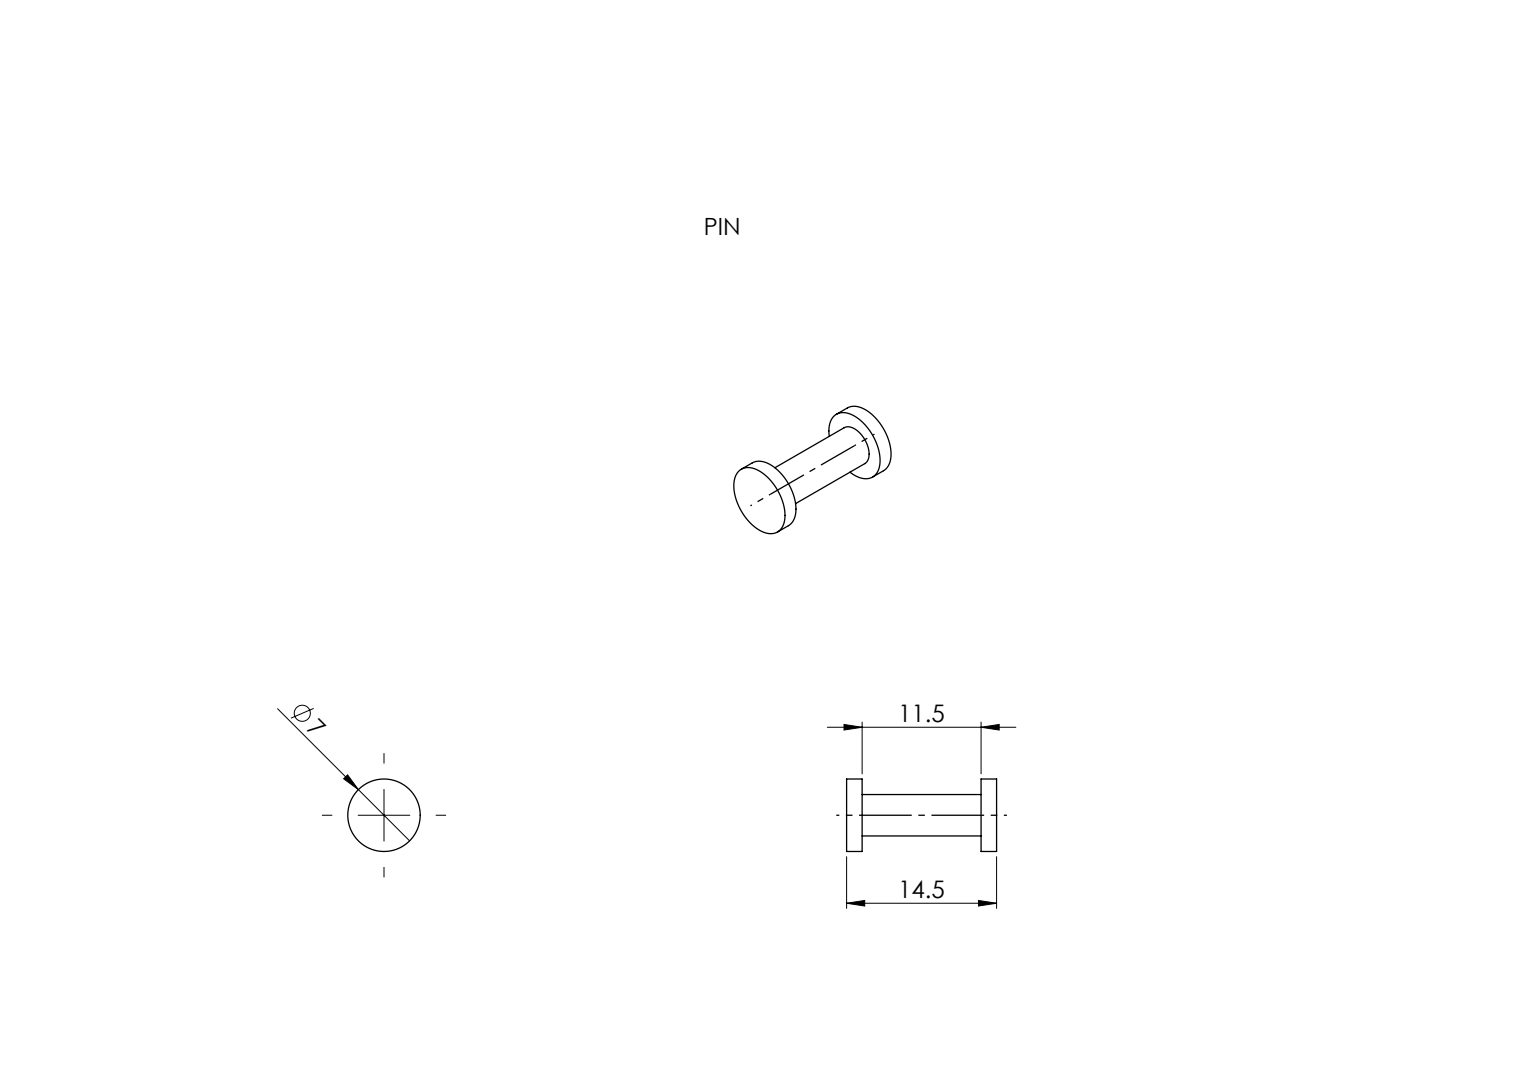
ISO-10303-21;
HEADER;
FILE_DESCRIPTION (('STEP AP214'),
    '1' );
FILE_NAME ('pin.step',
    '2026-10-08T13:56:24',
    ( '' ),
    ( '' ),
    'SwSTEP 2.0',
    'SolidWorks 2026',
    '' );
FILE_SCHEMA (( 'AUTOMOTIVE_DESIGN' ));
ENDSEC;

DATA;
#12=DIRECTION ( 'NONE',  ( 0.000000000000000000, 0.000000000000000000, 1.000000000000000000 ) ) ;
#38=ORIENTED_EDGE ( 'NONE', *, *, #402, .T. ) ;
#114=STYLED_ITEM ( 'NONE', ( #1544 ), #1156 ) ;
#128=FACE_OUTER_BOUND ( 'NONE', #6380, .T. ) ;
#244=CIRCLE ( 'NONE', #13904, 3.499999999999999556 ) ;
#268=ORIENTED_EDGE ( 'NONE', *, *, #2450, .T. ) ;
#279=SHAPE_REPRESENTATION ( 'pin', ( #3223 ), #1392 ) ;
#300=DIRECTION ( 'NONE',  ( 1.000000000000000000, 0.000000000000000000, 0.000000000000000000 ) ) ;
#402=EDGE_CURVE ( 'NONE', #3787, #10893, #14404, .T. ) ;
#420=ORIENTED_EDGE ( 'NONE', *, *, #9806, .F. ) ;
#470=AXIS2_PLACEMENT_3D ( 'NONE', #10148, #3841, #13765 ) ;
#493=AXIS2_PLACEMENT_3D ( 'NONE', #9026, #13762, #300 ) ;
#510=CYLINDRICAL_SURFACE ( 'NONE', #2443, 3.499999999999999556 ) ;
#545=ORIENTED_EDGE ( 'NONE', *, *, #14696, .T. ) ;
#561=ORIENTED_EDGE ( 'NONE', *, *, #4255, .T. ) ;
#598=ORIENTED_EDGE ( 'NONE', *, *, #1280, .F. ) ;
#604=CIRCLE ( 'NONE', #12193, 3.499999999999999556 ) ;
#652=DIRECTION ( 'NONE',  ( 0.000000000000000000, 0.000000000000000000, -1.000000000000000000 ) ) ;
#744=AXIS2_PLACEMENT_3D ( 'NONE', #6292, #7508, #3860 ) ;
#761=DIRECTION ( 'NONE',  ( 1.000000000000000000, 0.000000000000000000, 0.000000000000000000 ) ) ;
#824=PRESENTATION_STYLE_ASSIGNMENT (( #8512 ) ) ;
#867=EDGE_CURVE ( 'NONE', #14345, #10556, #6652, .T. ) ;
#971=FACE_OUTER_BOUND ( 'NONE', #5873, .T. ) ;
#1022=CARTESIAN_POINT ( 'NONE',  ( 16.49999999999956657, -8.786575603324269439E-13, 1.500000000000000000 ) ) ;
#1029=FACE_BOUND ( 'NONE', #10956, .T. ) ;
#1124=DIRECTION ( 'NONE',  ( 1.000000000000000000, 0.000000000000000000, -0.000000000000000000 ) ) ;
#1156=ADVANCED_BREP_SHAPE_REPRESENTATION ( '', ( #14368, #3223 ), #1392 ) ;
#1214=VERTEX_POINT ( 'NONE', #3633 ) ;
#1279=DIRECTION ( 'NONE',  ( 1.000000000000000000, 0.000000000000000000, 0.000000000000000000 ) ) ;
#1280=EDGE_CURVE ( 'NONE', #14345, #6321, #604, .T. ) ;
#1287=DIRECTION ( 'NONE',  ( 0.000000000000000000, 0.000000000000000000, 1.000000000000000000 ) ) ;
#1293=ORIENTED_EDGE ( 'NONE', *, *, #14089, .T. ) ;
#1392=( GEOMETRIC_REPRESENTATION_CONTEXT ( 3 ) GLOBAL_UNCERTAINTY_ASSIGNED_CONTEXT ( ( #13859 ) ) GLOBAL_UNIT_ASSIGNED_CONTEXT ( ( #13328, #11002, #7290 ) ) REPRESENTATION_CONTEXT ( 'NONE', 'WORKASPACE' ) );
#1399=EDGE_CURVE ( 'NONE', #3787, #13461, #8894, .T. ) ;
#1418=DIRECTION ( 'NONE',  ( -0.000000000000000000, -0.000000000000000000, 1.000000000000000000 ) ) ;
#1458=FACE_OUTER_BOUND ( 'NONE', #4862, .T. ) ;
#1544=PRESENTATION_STYLE_ASSIGNMENT (( #6858 ) ) ;
#1546=DIRECTION ( 'NONE',  ( -0.000000000000000000, -0.000000000000000000, -1.000000000000000000 ) ) ;
#1885=DIRECTION ( 'NONE',  ( 0.000000000000000000, 0.000000000000000000, 1.000000000000000000 ) ) ;
#1897=ADVANCED_FACE ( 'NONE', ( #3041 ), #4340, .T. ) ;
#1912=SURFACE_SIDE_STYLE ('',( #4264 ) ) ;
#2171=CARTESIAN_POINT ( 'NONE',  ( 19.99999999999956657, -8.786575603324269439E-13, -13.00000000000000000 ) ) ;
#2257=DIRECTION ( 'NONE',  ( -1.000000000000000000, 0.000000000000000000, 0.000000000000000000 ) ) ;
#2264=( NAMED_UNIT ( * ) SI_UNIT ( $, .STERADIAN. ) SOLID_ANGLE_UNIT ( ) );
#2282=PRODUCT ( 'pin', 'pin', '', ( #8596 ) ) ;
#2424=SHAPE_DEFINITION_REPRESENTATION ( #11948, #279 ) ;
#2431=AXIS2_PLACEMENT_3D ( 'NONE', #12948, #1885, #6826 ) ;
#2443=AXIS2_PLACEMENT_3D ( 'NONE', #2666, #1546, #7617 ) ;
#2450=EDGE_CURVE ( 'NONE', #10893, #1214, #15851, .T. ) ;
#2467=ADVANCED_FACE ( 'NONE', ( #14632, #8508 ), #7283, .F. ) ;
#2621=VERTEX_POINT ( 'NONE', #14297 ) ;
#2664=FILL_AREA_STYLE_COLOUR ( '', #3713 ) ;
#2666=CARTESIAN_POINT ( 'NONE',  ( 19.99999999999956657, -8.786575603324269439E-13, 1.500000000000000000 ) ) ;
#2707=COLOUR_RGB ( '', 0.72549020, 0.75294118, 0.79215686) ;
#2730=DIRECTION ( 'NONE',  ( -1.000000000000000000, 0.000000000000000000, 0.000000000000000000 ) ) ;
#2733=DIRECTION ( 'NONE',  ( 0.000000000000000000, 0.000000000000000000, 1.000000000000000000 ) ) ;
#2775=CIRCLE ( 'NONE', #12586, 3.499999999999999556 ) ;
#2780=APPLICATION_CONTEXT ( 'automotive_design' ) ;
#2797=CIRCLE ( 'NONE', #13897, 1.999999999999998224 ) ;
#2804=DIRECTION ( 'NONE',  ( 0.000000000000000000, 0.000000000000000000, 1.000000000000000000 ) ) ;
#2857=ORIENTED_EDGE ( 'NONE', *, *, #14089, .F. ) ;
#2908=DIRECTION ( 'NONE',  ( 0.000000000000000000, 0.000000000000000000, 1.000000000000000000 ) ) ;
#2968=CIRCLE ( 'NONE', #11735, 3.499999999999999556 ) ;
#3041=FACE_OUTER_BOUND ( 'NONE', #8493, .T. ) ;
#3057=( NAMED_UNIT ( * ) PLANE_ANGLE_UNIT ( ) SI_UNIT ( $, .RADIAN. ) );
#3115=EDGE_LOOP ( 'NONE', ( #5621, #10954 ) ) ;
#3133=VERTEX_POINT ( 'NONE', #5634 ) ;
#3171=VERTEX_POINT ( 'NONE', #11913 ) ;
#3223=AXIS2_PLACEMENT_3D ( 'NONE', #11897, #11972, #4638 ) ;
#3330=SURFACE_SIDE_STYLE ('',( #15617 ) ) ;
#3377=DIRECTION ( 'NONE',  ( 1.000000000000000000, 0.000000000000000000, 0.000000000000000000 ) ) ;
#3390=CARTESIAN_POINT ( 'NONE',  ( 19.99999999999956657, -8.786575603324269439E-13, 1.500000000000000000 ) ) ;
#3458=MECHANICAL_DESIGN_GEOMETRIC_PRESENTATION_REPRESENTATION('',(#114),#10179);
#3461=AXIS2_PLACEMENT_3D ( 'NONE', #12185, #1287, #1124 ) ;
#3471=( NAMED_UNIT ( * ) PLANE_ANGLE_UNIT ( ) SI_UNIT ( $, .RADIAN. ) );
#3501=CARTESIAN_POINT ( 'NONE',  ( 19.99999999999956657, -8.786575603324269439E-13, -11.50000000000000000 ) ) ;
#3633=CARTESIAN_POINT ( 'NONE',  ( 17.99999999999957012, -8.784126309725975241E-13, 0.000000000000000000 ) ) ;
#3688=DIRECTION ( 'NONE',  ( 0.000000000000000000, 0.000000000000000000, 1.000000000000000000 ) ) ;
#3702=DIRECTION ( 'NONE',  ( 1.000000000000000000, 0.000000000000000000, -0.000000000000000000 ) ) ;
#3713=COLOUR_RGB ( '', 0.72549020, 0.75294118, 0.79215686) ;
#3724=CARTESIAN_POINT ( 'NONE',  ( 19.99999999999956657, -8.786575603324269439E-13, -13.00000000000000000 ) ) ;
#3734=ORIENTED_EDGE ( 'NONE', *, *, #14085, .T. ) ;
#3787=VERTEX_POINT ( 'NONE', #14980 ) ;
#3835=VECTOR ( 'NONE', #8593, 1000.000000000000000 ) ;
#3841=DIRECTION ( 'NONE',  ( -0.000000000000000000, -0.000000000000000000, -1.000000000000000000 ) ) ;
#3860=DIRECTION ( 'NONE',  ( 1.000000000000000000, 0.000000000000000000, 0.000000000000000000 ) ) ;
#4016=AXIS2_PLACEMENT_3D ( 'NONE', #2171, #8417, #1279 ) ;
#4126=EDGE_LOOP ( 'NONE', ( #598, #10600, #4186, #11155 ) ) ;
#4148=PRODUCT_DEFINITION_CONTEXT ( 'detailed design', #2780, 'design' ) ;
#4186=ORIENTED_EDGE ( 'NONE', *, *, #9806, .T. ) ;
#4255=EDGE_CURVE ( 'NONE', #13119, #10556, #13568, .T. ) ;
#4264=SURFACE_STYLE_FILL_AREA ( #7536 ) ;
#4340=CYLINDRICAL_SURFACE ( 'NONE', #7830, 1.999999999999998224 ) ;
#4360=ADVANCED_FACE ( 'NONE', ( #1029, #12326 ), #5964, .F. ) ;
#4374=ORIENTED_EDGE ( 'NONE', *, *, #7133, .T. ) ;
#4468=CARTESIAN_POINT ( 'NONE',  ( 16.49999999999956657, -8.786575603324269439E-13, 1.500000000000000000 ) ) ;
#4638=DIRECTION ( 'NONE',  ( 1.000000000000000000, 0.000000000000000000, 0.000000000000000000 ) ) ;
#4640=ORIENTED_EDGE ( 'NONE', *, *, #4912, .F. ) ;
#4744=CARTESIAN_POINT ( 'NONE',  ( 19.99999999999956657, -8.786575603324269439E-13, -11.50000000000000000 ) ) ;
#4827=CARTESIAN_POINT ( 'NONE',  ( 19.99999999999956657, -8.786575603324269439E-13, -11.50000000000000000 ) ) ;
#4862=EDGE_LOOP ( 'NONE', ( #9433, #4374, #9993, #8827 ) ) ;
#4902=EDGE_LOOP ( 'NONE', ( #6854, #14386 ) ) ;
#4906=DIRECTION ( 'NONE',  ( 0.000000000000000000, 0.000000000000000000, -1.000000000000000000 ) ) ;
#4912=EDGE_CURVE ( 'NONE', #10893, #3787, #8460, .T. ) ;
#5022=LINE ( 'NONE', #13484, #3835 ) ;
#5101=( NAMED_UNIT ( * ) SI_UNIT ( $, .STERADIAN. ) SOLID_ANGLE_UNIT ( ) );
#5151=DIRECTION ( 'NONE',  ( 0.000000000000000000, 0.000000000000000000, 1.000000000000000000 ) ) ;
#5508=ORIENTED_EDGE ( 'NONE', *, *, #7307, .F. ) ;
#5576=DIRECTION ( 'NONE',  ( -1.000000000000000000, 0.000000000000000000, 0.000000000000000000 ) ) ;
#5621=ORIENTED_EDGE ( 'NONE', *, *, #8865, .F. ) ;
#5634=CARTESIAN_POINT ( 'NONE',  ( 23.49999999999956657, -8.782289339527253835E-13, 1.500000000000000000 ) ) ;
#5873=EDGE_LOOP ( 'NONE', ( #1293, #545 ) ) ;
#5964=PLANE ( 'NONE',  #12294 ) ;
#6005=ADVANCED_FACE ( 'NONE', ( #8859 ), #6589, .T. ) ;
#6166=PLANE ( 'NONE',  #8962 ) ;
#6209=DIRECTION ( 'NONE',  ( -1.000000000000000000, 0.000000000000000000, 0.000000000000000000 ) ) ;
#6225=FACE_OUTER_BOUND ( 'NONE', #4126, .T. ) ;
#6292=CARTESIAN_POINT ( 'NONE',  ( 19.99999999999956657, -8.786575603324269439E-13, 0.000000000000000000 ) ) ;
#6320=CARTESIAN_POINT ( 'NONE',  ( 19.99999999999956657, -8.786575603324269439E-13, 0.000000000000000000 ) ) ;
#6321=VERTEX_POINT ( 'NONE', #14810 ) ;
#6380=EDGE_LOOP ( 'NONE', ( #8663, #11359, #11699, #561 ) ) ;
#6403=ORIENTED_EDGE ( 'NONE', *, *, #8676, .T. ) ;
#6481=( LENGTH_UNIT ( ) NAMED_UNIT ( * ) SI_UNIT ( .MILLI., .METRE. ) );
#6521=CARTESIAN_POINT ( 'NONE',  ( 23.49999999999956657, -8.786575603324269439E-13, -13.00000000000000000 ) ) ;
#6589=CYLINDRICAL_SURFACE ( 'NONE', #470, 3.499999999999999556 ) ;
#6652=LINE ( 'NONE', #8997, #15308 ) ;
#6732=ORIENTED_EDGE ( 'NONE', *, *, #1399, .T. ) ;
#6767=DIRECTION ( 'NONE',  ( 1.000000000000000000, 0.000000000000000000, 0.000000000000000000 ) ) ;
#6821=DIRECTION ( 'NONE',  ( 0.000000000000000000, 0.000000000000000000, 1.000000000000000000 ) ) ;
#6826=DIRECTION ( 'NONE',  ( 1.000000000000000000, 0.000000000000000000, 0.000000000000000000 ) ) ;
#6835=VECTOR ( 'NONE', #12, 1000.000000000000000 ) ;
#6854=ORIENTED_EDGE ( 'NONE', *, *, #7307, .T. ) ;
#6858=SURFACE_STYLE_USAGE ( .BOTH. , #1912 ) ;
#6874=AXIS2_PLACEMENT_3D ( 'NONE', #3390, #15842, #3702 ) ;
#7006=EDGE_CURVE ( 'NONE', #1214, #13461, #2797, .T. ) ;
#7008=DIRECTION ( 'NONE',  ( 0.000000000000000000, 0.000000000000000000, 1.000000000000000000 ) ) ;
#7112=CIRCLE ( 'NONE', #2431, 3.499999999999999556 ) ;
#7120=PLANE ( 'NONE',  #6874 ) ;
#7133=EDGE_CURVE ( 'NONE', #3133, #3171, #5022, .T. ) ;
#7283=PLANE ( 'NONE',  #3461 ) ;
#7290=( NAMED_UNIT ( * ) SI_UNIT ( $, .STERADIAN. ) SOLID_ANGLE_UNIT ( ) );
#7307=EDGE_CURVE ( 'NONE', #13461, #1214, #10305, .T. ) ;
#7442=DIRECTION ( 'NONE',  ( 0.000000000000000000, 0.000000000000000000, -1.000000000000000000 ) ) ;
#7508=DIRECTION ( 'NONE',  ( 0.000000000000000000, 0.000000000000000000, 1.000000000000000000 ) ) ;
#7536=FILL_AREA_STYLE ('',( #2664 ) ) ;
#7617=DIRECTION ( 'NONE',  ( -1.000000000000000000, 0.000000000000000000, 0.000000000000000000 ) ) ;
#7655=ORIENTED_EDGE ( 'NONE', *, *, #1280, .T. ) ;
#7830=AXIS2_PLACEMENT_3D ( 'NONE', #13043, #7008, #6767 ) ;
#7897=CARTESIAN_POINT ( 'NONE',  ( 19.99999999999956657, -8.786575603324269439E-13, -11.50000000000000000 ) ) ;
#7961=LINE ( 'NONE', #4468, #8160 ) ;
#8160=VECTOR ( 'NONE', #10544, 1000.000000000000000 ) ;
#8186=CLOSED_SHELL ( 'NONE', ( #11457, #11195, #1897, #8884, #6005, #11456, #2467, #9196, #12602, #4360 ) ) ;
#8379=DIRECTION ( 'NONE',  ( 1.000000000000000000, 0.000000000000000000, 0.000000000000000000 ) ) ;
#8417=DIRECTION ( 'NONE',  ( -0.000000000000000000, -0.000000000000000000, 1.000000000000000000 ) ) ;
#8460=CIRCLE ( 'NONE', #9479, 1.999999999999998224 ) ;
#8493=EDGE_LOOP ( 'NONE', ( #38, #268, #5508, #11280 ) ) ;
#8508=FACE_OUTER_BOUND ( 'NONE', #3115, .T. ) ;
#8512=SURFACE_STYLE_USAGE ( .BOTH. , #3330 ) ;
#8593=DIRECTION ( 'NONE',  ( -0.000000000000000000, -0.000000000000000000, -1.000000000000000000 ) ) ;
#8596=PRODUCT_CONTEXT ( 'NONE', #14240, 'mechanical' ) ;
#8633=DIRECTION ( 'NONE',  ( 0.000000000000000000, 0.000000000000000000, -1.000000000000000000 ) ) ;
#8663=ORIENTED_EDGE ( 'NONE', *, *, #867, .F. ) ;
#8676=EDGE_CURVE ( 'NONE', #6321, #14345, #2775, .T. ) ;
#8719=FACE_OUTER_BOUND ( 'NONE', #14361, .T. ) ;
#8827=ORIENTED_EDGE ( 'NONE', *, *, #14085, .F. ) ;
#8859=FACE_OUTER_BOUND ( 'NONE', #11536, .T. ) ;
#8865=EDGE_CURVE ( 'NONE', #2621, #3171, #13356, .T. ) ;
#8884=ADVANCED_FACE ( 'NONE', ( #8719 ), #13625, .T. ) ;
#8894=LINE ( 'NONE', #13796, #15576 ) ;
#8962=AXIS2_PLACEMENT_3D ( 'NONE', #3724, #14431, #13192 ) ;
#8997=CARTESIAN_POINT ( 'NONE',  ( 16.49999999999956657, -8.782289339527253835E-13, -13.00000000000000000 ) ) ;
#9026=CARTESIAN_POINT ( 'NONE',  ( 19.99999999999956657, -8.786575603324269439E-13, -13.00000000000000000 ) ) ;
#9092=CARTESIAN_POINT ( 'NONE',  ( 19.99999999999956657, -8.786575603324269439E-13, 1.500000000000000000 ) ) ;
#9126=ORIENTED_EDGE ( 'NONE', *, *, #8865, .T. ) ;
#9173=STYLED_ITEM ( 'NONE', ( #824 ), #14368 ) ;
#9196=ADVANCED_FACE ( 'NONE', ( #128 ), #11112, .T. ) ;
#9220=CARTESIAN_POINT ( 'NONE',  ( 19.99999999999956657, -8.786575603324269439E-13, -13.00000000000000000 ) ) ;
#9304=EDGE_LOOP ( 'NONE', ( #13905, #420 ) ) ;
#9393=FILL_AREA_STYLE_COLOUR ( '', #2707 ) ;
#9433=ORIENTED_EDGE ( 'NONE', *, *, #14696, .F. ) ;
#9468=AXIS2_PLACEMENT_3D ( 'NONE', #4827, #8633, #6209 ) ;
#9479=AXIS2_PLACEMENT_3D ( 'NONE', #3501, #9730, #8379 ) ;
#9690=DIRECTION ( 'NONE',  ( 0.000000000000000000, 0.000000000000000000, -1.000000000000000000 ) ) ;
#9730=DIRECTION ( 'NONE',  ( 0.000000000000000000, 0.000000000000000000, 1.000000000000000000 ) ) ;
#9794=ORIENTED_EDGE ( 'NONE', *, *, #2450, .F. ) ;
#9806=EDGE_CURVE ( 'NONE', #10556, #13119, #244, .T. ) ;
#9989=PRODUCT_DEFINITION_FORMATION_WITH_SPECIFIED_SOURCE ( 'ANY', '', #2282, .NOT_KNOWN. ) ;
#9993=ORIENTED_EDGE ( 'NONE', *, *, #11179, .T. ) ;
#10026=CARTESIAN_POINT ( 'NONE',  ( 17.99999999999957012, -8.784126309725975241E-13, -11.50000000000000000 ) ) ;
#10080=DIRECTION ( 'NONE',  ( 1.000000000000000000, 0.000000000000000000, 0.000000000000000000 ) ) ;
#10119=DIRECTION ( 'NONE',  ( -0.000000000000000000, -0.000000000000000000, 1.000000000000000000 ) ) ;
#10148=CARTESIAN_POINT ( 'NONE',  ( 19.99999999999956657, -8.786575603324269439E-13, 1.500000000000000000 ) ) ;
#10179=( GEOMETRIC_REPRESENTATION_CONTEXT ( 3 ) GLOBAL_UNCERTAINTY_ASSIGNED_CONTEXT ( ( #12702 ) ) GLOBAL_UNIT_ASSIGNED_CONTEXT ( ( #6481, #3057, #5101 ) ) REPRESENTATION_CONTEXT ( 'NONE', 'WORKASPACE' ) );
#10182=CARTESIAN_POINT ( 'NONE',  ( 19.99999999999956657, -8.786575603324269439E-13, -11.50000000000000000 ) ) ;
#10285=DIRECTION ( 'NONE',  ( 1.000000000000000000, 0.000000000000000000, 0.000000000000000000 ) ) ;
#10305=CIRCLE ( 'NONE', #14687, 1.999999999999998224 ) ;
#10410=ORIENTED_EDGE ( 'NONE', *, *, #402, .F. ) ;
#10544=DIRECTION ( 'NONE',  ( -0.000000000000000000, -0.000000000000000000, -1.000000000000000000 ) ) ;
#10556=VERTEX_POINT ( 'NONE', #15643 ) ;
#10600=ORIENTED_EDGE ( 'NONE', *, *, #867, .T. ) ;
#10893=VERTEX_POINT ( 'NONE', #14250 ) ;
#10912=FILL_AREA_STYLE ('',( #9393 ) ) ;
#10954=ORIENTED_EDGE ( 'NONE', *, *, #11179, .F. ) ;
#10956=EDGE_LOOP ( 'NONE', ( #10410, #4640 ) ) ;
#10967=CARTESIAN_POINT ( 'NONE',  ( 19.99999999999956657, -8.786575603324269439E-13, 0.000000000000000000 ) ) ;
#10976=MECHANICAL_DESIGN_GEOMETRIC_PRESENTATION_REPRESENTATION('',(#9173),#11981);
#11002=( NAMED_UNIT ( * ) PLANE_ANGLE_UNIT ( ) SI_UNIT ( $, .RADIAN. ) );
#11112=CYLINDRICAL_SURFACE ( 'NONE', #493, 3.499999999999999556 ) ;
#11155=ORIENTED_EDGE ( 'NONE', *, *, #13618, .F. ) ;
#11179=EDGE_CURVE ( 'NONE', #3171, #2621, #12772, .T. ) ;
#11195=ADVANCED_FACE ( 'NONE', ( #1458 ), #510, .T. ) ;
#11280=ORIENTED_EDGE ( 'NONE', *, *, #1399, .F. ) ;
#11359=ORIENTED_EDGE ( 'NONE', *, *, #8676, .F. ) ;
#11456=ADVANCED_FACE ( 'NONE', ( #971 ), #7120, .T. ) ;
#11457=ADVANCED_FACE ( 'NONE', ( #6225 ), #13231, .T. ) ;
#11536=EDGE_LOOP ( 'NONE', ( #13078, #2857, #3734, #9126 ) ) ;
#11628=EDGE_LOOP ( 'NONE', ( #6403, #7655 ) ) ;
#11699=ORIENTED_EDGE ( 'NONE', *, *, #13618, .T. ) ;
#11726=VECTOR ( 'NONE', #1418, 1000.000000000000000 ) ;
#11735=AXIS2_PLACEMENT_3D ( 'NONE', #9092, #13018, #761 ) ;
#11897=CARTESIAN_POINT ( 'NONE',  ( 0.000000000000000000, 0.000000000000000000, 0.000000000000000000 ) ) ;
#11913=CARTESIAN_POINT ( 'NONE',  ( 23.49999999999956657, -8.782289339527253835E-13, 0.000000000000000000 ) ) ;
#11948=PRODUCT_DEFINITION_SHAPE ( 'NONE', 'NONE',  #13413 ) ;
#11972=DIRECTION ( 'NONE',  ( 0.000000000000000000, 0.000000000000000000, 1.000000000000000000 ) ) ;
#11981=( GEOMETRIC_REPRESENTATION_CONTEXT ( 3 ) GLOBAL_UNCERTAINTY_ASSIGNED_CONTEXT ( ( #15507 ) ) GLOBAL_UNIT_ASSIGNED_CONTEXT ( ( #15700, #3471, #2264 ) ) REPRESENTATION_CONTEXT ( 'NONE', 'WORKASPACE' ) );
#12004=CARTESIAN_POINT ( 'NONE',  ( 21.99999999999956657, -8.786575603324269439E-13, 0.000000000000000000 ) ) ;
#12185=CARTESIAN_POINT ( 'NONE',  ( 19.99999999999956657, -8.786575603324269439E-13, 0.000000000000000000 ) ) ;
#12193=AXIS2_PLACEMENT_3D ( 'NONE', #13315, #9690, #2257 ) ;
#12294=AXIS2_PLACEMENT_3D ( 'NONE', #4744, #4906, #13378 ) ;
#12326=FACE_OUTER_BOUND ( 'NONE', #9304, .T. ) ;
#12439=ORIENTED_EDGE ( 'NONE', *, *, #4912, .T. ) ;
#12586=AXIS2_PLACEMENT_3D ( 'NONE', #9220, #652, #5576 ) ;
#12602=ADVANCED_FACE ( 'NONE', ( #15647 ), #6166, .T. ) ;
#12645=LINE ( 'NONE', #6521, #11726 ) ;
#12702=UNCERTAINTY_MEASURE_WITH_UNIT (LENGTH_MEASURE( 1.000000000000000082E-05 ), #6481, 'distance_accuracy_value', 'NONE');
#12772=CIRCLE ( 'NONE', #13540, 3.499999999999999556 ) ;
#12948=CARTESIAN_POINT ( 'NONE',  ( 19.99999999999956657, -8.786575603324269439E-13, 1.500000000000000000 ) ) ;
#13018=DIRECTION ( 'NONE',  ( 0.000000000000000000, 0.000000000000000000, 1.000000000000000000 ) ) ;
#13043=CARTESIAN_POINT ( 'NONE',  ( 19.99999999999956657, -8.786575603324269439E-13, -11.50000000000000000 ) ) ;
#13078=ORIENTED_EDGE ( 'NONE', *, *, #7133, .F. ) ;
#13103=DIRECTION ( 'NONE',  ( 1.000000000000000000, 0.000000000000000000, 0.000000000000000000 ) ) ;
#13119=VERTEX_POINT ( 'NONE', #13638 ) ;
#13192=DIRECTION ( 'NONE',  ( -1.000000000000000000, 0.000000000000000000, -0.000000000000000000 ) ) ;
#13231=CYLINDRICAL_SURFACE ( 'NONE', #4016, 3.499999999999999556 ) ;
#13315=CARTESIAN_POINT ( 'NONE',  ( 19.99999999999956657, -8.786575603324269439E-13, -13.00000000000000000 ) ) ;
#13328=( LENGTH_UNIT ( ) NAMED_UNIT ( * ) SI_UNIT ( .MILLI., .METRE. ) );
#13356=CIRCLE ( 'NONE', #744, 3.499999999999999556 ) ;
#13378=DIRECTION ( 'NONE',  ( -1.000000000000000000, 0.000000000000000000, -0.000000000000000000 ) ) ;
#13411=CARTESIAN_POINT ( 'NONE',  ( 16.49999999999956657, -8.782289339527253835E-13, -13.00000000000000000 ) ) ;
#13413=PRODUCT_DEFINITION ( 'UNKNOWN', '', #9989, #4148 ) ;
#13461=VERTEX_POINT ( 'NONE', #12004 ) ;
#13484=CARTESIAN_POINT ( 'NONE',  ( 23.49999999999956657, -8.782289339527253835E-13, 1.500000000000000000 ) ) ;
#13540=AXIS2_PLACEMENT_3D ( 'NONE', #6320, #2908, #10285 ) ;
#13568=CIRCLE ( 'NONE', #9468, 3.499999999999999556 ) ;
#13618=EDGE_CURVE ( 'NONE', #6321, #13119, #12645, .T. ) ;
#13625=CYLINDRICAL_SURFACE ( 'NONE', #14664, 1.999999999999998224 ) ;
#13638=CARTESIAN_POINT ( 'NONE',  ( 23.49999999999956657, -8.786575603324269439E-13, -11.50000000000000000 ) ) ;
#13762=DIRECTION ( 'NONE',  ( -0.000000000000000000, -0.000000000000000000, 1.000000000000000000 ) ) ;
#13765=DIRECTION ( 'NONE',  ( -1.000000000000000000, 0.000000000000000000, 0.000000000000000000 ) ) ;
#13796=CARTESIAN_POINT ( 'NONE',  ( 21.99999999999956657, -8.786575603324269439E-13, -11.50000000000000000 ) ) ;
#13810=SHAPE_REPRESENTATION_RELATIONSHIP ( 'NONE' , 'NONE' ,  #279, #1156 ) ;
#13859=UNCERTAINTY_MEASURE_WITH_UNIT (LENGTH_MEASURE( 1.000000000000000082E-05 ), #13328, 'distance_accuracy_value', 'NONE');
#13871=CARTESIAN_POINT ( 'NONE',  ( 19.99999999999956657, -8.786575603324269439E-13, -11.50000000000000000 ) ) ;
#13897=AXIS2_PLACEMENT_3D ( 'NONE', #15553, #6821, #13103 ) ;
#13904=AXIS2_PLACEMENT_3D ( 'NONE', #10182, #7442, #2730 ) ;
#13905=ORIENTED_EDGE ( 'NONE', *, *, #4255, .F. ) ;
#14085=EDGE_CURVE ( 'NONE', #15535, #2621, #7961, .T. ) ;
#14089=EDGE_CURVE ( 'NONE', #15535, #3133, #2968, .T. ) ;
#14240=APPLICATION_CONTEXT ( 'automotive_design' ) ;
#14250=CARTESIAN_POINT ( 'NONE',  ( 17.99999999999957012, -8.784126309725975241E-13, -11.50000000000000000 ) ) ;
#14297=CARTESIAN_POINT ( 'NONE',  ( 16.49999999999956657, -8.786575603324269439E-13, 0.000000000000000000 ) ) ;
#14345=VERTEX_POINT ( 'NONE', #13411 ) ;
#14361=EDGE_LOOP ( 'NONE', ( #9794, #12439, #6732, #14461 ) ) ;
#14368=MANIFOLD_SOLID_BREP ( 'Boss-Extrude3', #8186 ) ;
#14386=ORIENTED_EDGE ( 'NONE', *, *, #7006, .T. ) ;
#14404=CIRCLE ( 'NONE', #15175, 1.999999999999998224 ) ;
#14431=DIRECTION ( 'NONE',  ( 0.000000000000000000, 0.000000000000000000, -1.000000000000000000 ) ) ;
#14461=ORIENTED_EDGE ( 'NONE', *, *, #7006, .F. ) ;
#14632=FACE_BOUND ( 'NONE', #4902, .T. ) ;
#14664=AXIS2_PLACEMENT_3D ( 'NONE', #13871, #2804, #15017 ) ;
#14687=AXIS2_PLACEMENT_3D ( 'NONE', #10967, #3688, #3377 ) ;
#14696=EDGE_CURVE ( 'NONE', #3133, #15535, #7112, .T. ) ;
#14810=CARTESIAN_POINT ( 'NONE',  ( 23.49999999999956657, -8.786575603324269439E-13, -13.00000000000000000 ) ) ;
#14980=CARTESIAN_POINT ( 'NONE',  ( 21.99999999999956657, -8.786575603324269439E-13, -11.50000000000000000 ) ) ;
#15017=DIRECTION ( 'NONE',  ( 1.000000000000000000, 0.000000000000000000, 0.000000000000000000 ) ) ;
#15175=AXIS2_PLACEMENT_3D ( 'NONE', #7897, #5151, #10080 ) ;
#15308=VECTOR ( 'NONE', #10119, 1000.000000000000000 ) ;
#15507=UNCERTAINTY_MEASURE_WITH_UNIT (LENGTH_MEASURE( 1.000000000000000082E-05 ), #15700, 'distance_accuracy_value', 'NONE');
#15535=VERTEX_POINT ( 'NONE', #1022 ) ;
#15553=CARTESIAN_POINT ( 'NONE',  ( 19.99999999999956657, -8.786575603324269439E-13, 0.000000000000000000 ) ) ;
#15576=VECTOR ( 'NONE', #2733, 1000.000000000000000 ) ;
#15617=SURFACE_STYLE_FILL_AREA ( #10912 ) ;
#15643=CARTESIAN_POINT ( 'NONE',  ( 16.49999999999956657, -8.782289339527253835E-13, -11.50000000000000000 ) ) ;
#15647=FACE_OUTER_BOUND ( 'NONE', #11628, .T. ) ;
#15700=( LENGTH_UNIT ( ) NAMED_UNIT ( * ) SI_UNIT ( .MILLI., .METRE. ) );
#15842=DIRECTION ( 'NONE',  ( 0.000000000000000000, 0.000000000000000000, 1.000000000000000000 ) ) ;
#15851=LINE ( 'NONE', #10026, #6835 ) ;
ENDSEC;
END-ISO-10303-21;
